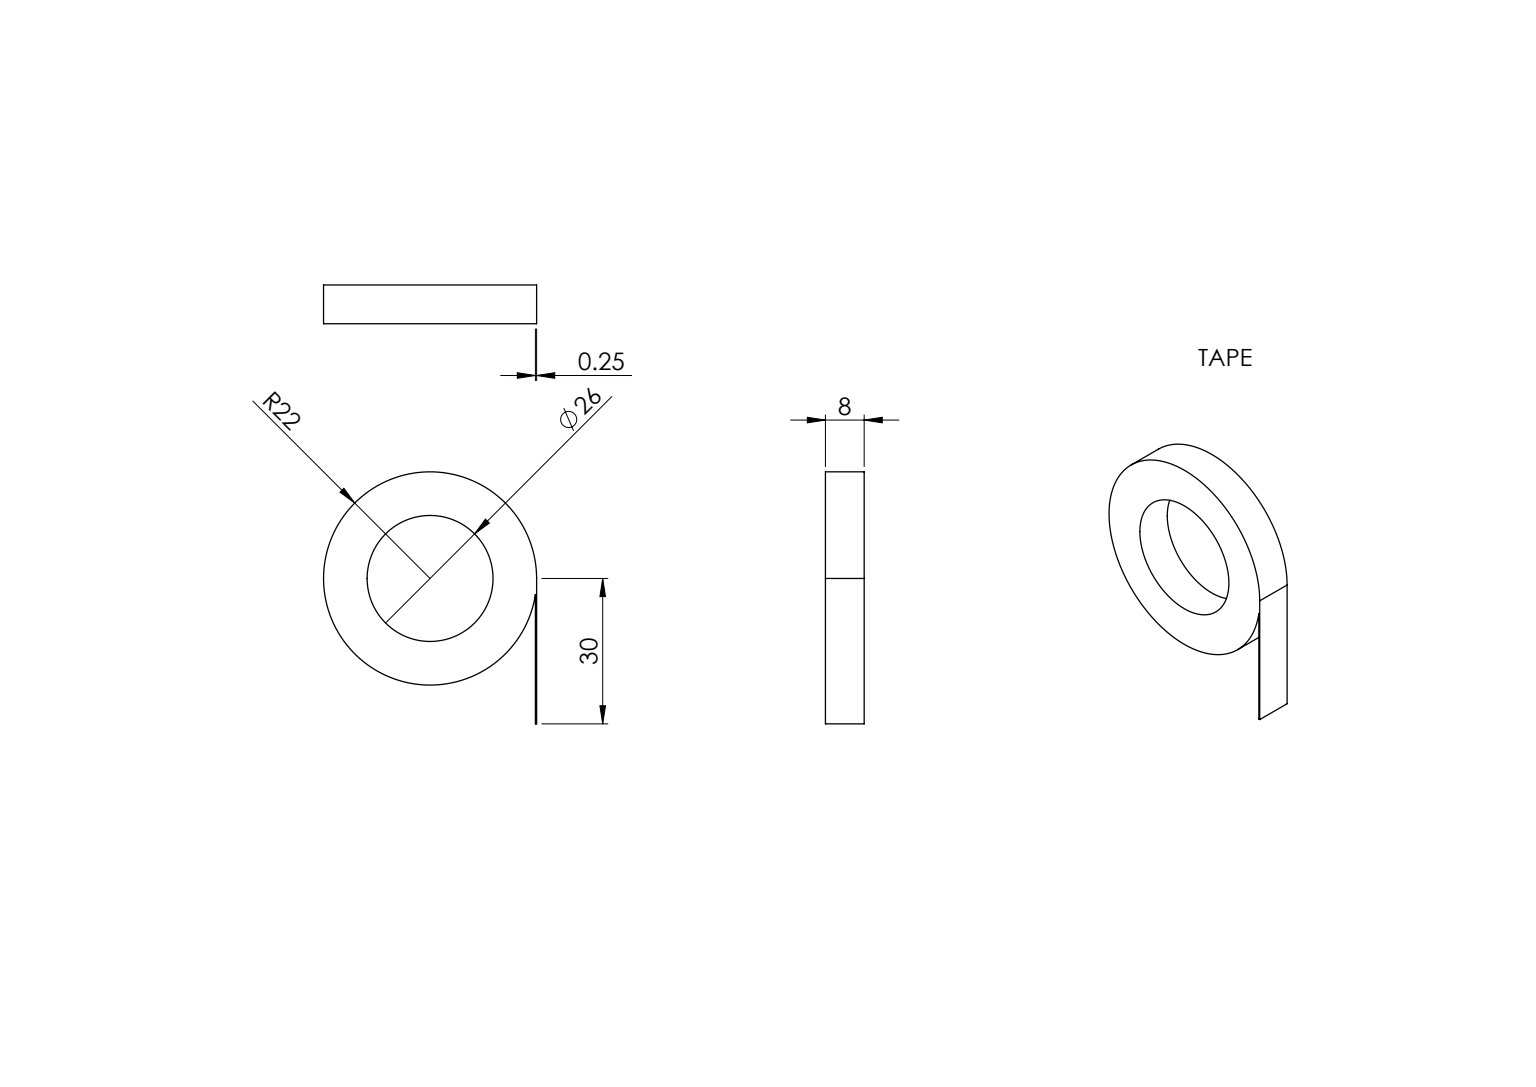
ISO-10303-21;
HEADER;
FILE_DESCRIPTION (('STEP AP214'),
    '1' );
FILE_NAME ('tape.step',
    '2026-10-23T14:45:25',
    ( '' ),
    ( '' ),
    'SwSTEP 2.0',
    'SolidWorks 2026',
    '' );
FILE_SCHEMA (( 'AUTOMOTIVE_DESIGN' ));
ENDSEC;

DATA;
#10=FACE_OUTER_BOUND ( 'NONE', #593, .T. ) ;
#25=LINE ( 'NONE', #396, #4267 ) ;
#41=DIRECTION ( 'NONE',  ( -0.000000000000000000, -0.000000000000000000, 1.000000000000000000 ) ) ;
#112=FACE_OUTER_BOUND ( 'NONE', #2425, .T. ) ;
#144=AXIS2_PLACEMENT_3D ( 'NONE', #2084, #4329, #2630 ) ;
#147=VECTOR ( 'NONE', #3798, 1000.000000000000000 ) ;
#160=DIRECTION ( 'NONE',  ( -1.000000000000000000, 1.156482317317871478E-16, 0.000000000000000000 ) ) ;
#169=FILL_AREA_STYLE ('',( #1465 ) ) ;
#177=PRODUCT_DEFINITION ( 'UNKNOWN', '', #2504, #5623 ) ;
#186=VERTEX_POINT ( 'NONE', #5039 ) ;
#263=FACE_OUTER_BOUND ( 'NONE', #5640, .T. ) ;
#276=VERTEX_POINT ( 'NONE', #4778 ) ;
#281=CARTESIAN_POINT ( 'NONE',  ( 21.74999999999999645, -30.00000000000000000, 4.000000000000001776 ) ) ;
#283=CARTESIAN_POINT ( 'NONE',  ( 0.000000000000000000, 0.000000000000000000, 0.000000000000000000 ) ) ;
#300=VERTEX_POINT ( 'NONE', #812 ) ;
#317=CARTESIAN_POINT ( 'NONE',  ( 21.74999999999999645, -30.00000000000000000, 4.000000000000001776 ) ) ;
#322=AXIS2_PLACEMENT_3D ( 'NONE', #2249, #3206, #3094 ) ;
#341=DIRECTION ( 'NONE',  ( -0.000000000000000000, -0.000000000000000000, 1.000000000000000000 ) ) ;
#377=ORIENTED_EDGE ( 'NONE', *, *, #2965, .T. ) ;
#391=PRODUCT_CONTEXT ( 'NONE', #2359, 'mechanical' ) ;
#396=CARTESIAN_POINT ( 'NONE',  ( 22.00000000000000000, 0.000000000000000000, 4.000000000000001776 ) ) ;
#443=EDGE_LOOP ( 'NONE', ( #3408, #675, #377, #4015 ) ) ;
#514=DIRECTION ( 'NONE',  ( -1.156482317317871478E-16, -1.000000000000000000, 0.000000000000000000 ) ) ;
#593=EDGE_LOOP ( 'NONE', ( #4807, #5299, #2400, #5252 ) ) ;
#599=SURFACE_STYLE_USAGE ( .BOTH. , #3222 ) ;
#602=ORIENTED_EDGE ( 'NONE', *, *, #3162, .F. ) ;
#606=CIRCLE ( 'NONE', #4005, 22.00000000000000000 ) ;
#675=ORIENTED_EDGE ( 'NONE', *, *, #3739, .T. ) ;
#687=EDGE_CURVE ( 'NONE', #2844, #5686, #1361, .T. ) ;
#701=AXIS2_PLACEMENT_3D ( 'NONE', #1249, #817, #1709 ) ;
#717=VECTOR ( 'NONE', #3845, 1000.000000000000000 ) ;
#720=AXIS2_PLACEMENT_3D ( 'NONE', #2496, #3826, #4630 ) ;
#723=CARTESIAN_POINT ( 'NONE',  ( 0.000000000000000000, 0.000000000000000000, 12.00000000000000000 ) ) ;
#764=ADVANCED_FACE ( 'NONE', ( #112 ), #4631, .F. ) ;
#772=LINE ( 'NONE', #281, #3560 ) ;
#809=CARTESIAN_POINT ( 'NONE',  ( 21.75000000000000000, -3.307189138830739061, -58.22539674441618018 ) ) ;
#812=CARTESIAN_POINT ( 'NONE',  ( 21.99999999999999645, -30.00000000000000000, 4.000000000000001776 ) ) ;
#817=DIRECTION ( 'NONE',  ( 0.000000000000000000, 0.000000000000000000, -1.000000000000000000 ) ) ;
#829=SHAPE_DEFINITION_REPRESENTATION ( #2987, #1911 ) ;
#843=ORIENTED_EDGE ( 'NONE', *, *, #1114, .T. ) ;
#861=LINE ( 'NONE', #5267, #1138 ) ;
#905=CARTESIAN_POINT ( 'NONE',  ( -13.00000000000000178, 1.592040838891559293E-15, -58.22539674441618018 ) ) ;
#907=EDGE_LOOP ( 'NONE', ( #5557, #3894 ) ) ;
#947=CARTESIAN_POINT ( 'NONE',  ( -13.00000000000000178, 1.592040838891559293E-15, 12.00000000000000000 ) ) ;
#949=CARTESIAN_POINT ( 'NONE',  ( 21.74999999999999645, -30.00000000000000000, 12.00000000000000000 ) ) ;
#998=ADVANCED_FACE ( 'NONE', ( #2029 ), #2922, .F. ) ;
#1031=DIRECTION ( 'NONE',  ( -0.000000000000000000, -0.000000000000000000, 1.000000000000000000 ) ) ;
#1035=ORIENTED_EDGE ( 'NONE', *, *, #4653, .T. ) ;
#1070=DIRECTION ( 'NONE',  ( 0.000000000000000000, -0.000000000000000000, -1.000000000000000000 ) ) ;
#1094=EDGE_CURVE ( 'NONE', #300, #5686, #5596, .T. ) ;
#1114=EDGE_CURVE ( 'NONE', #5601, #276, #2089, .T. ) ;
#1138=VECTOR ( 'NONE', #3169, 1000.000000000000000 ) ;
#1148=AXIS2_PLACEMENT_3D ( 'NONE', #5005, #4577, #2387 ) ;
#1173=ORIENTED_EDGE ( 'NONE', *, *, #1220, .F. ) ;
#1220=EDGE_CURVE ( 'NONE', #186, #300, #4785, .T. ) ;
#1249=CARTESIAN_POINT ( 'NONE',  ( 0.000000000000000000, 0.000000000000000000, 4.000000000000000000 ) ) ;
#1282=FACE_OUTER_BOUND ( 'NONE', #5045, .T. ) ;
#1299=DIRECTION ( 'NONE',  ( 0.000000000000000000, 0.000000000000000000, -1.000000000000000000 ) ) ;
#1311=CARTESIAN_POINT ( 'NONE',  ( 13.00000000000000178, 0.000000000000000000, -58.22539674441618018 ) ) ;
#1312=MECHANICAL_DESIGN_GEOMETRIC_PRESENTATION_REPRESENTATION('',(#4977),#2871);
#1330=DIRECTION ( 'NONE',  ( -1.156482317317871725E-16, -1.000000000000000000, 0.000000000000000000 ) ) ;
#1333=VERTEX_POINT ( 'NONE', #5245 ) ;
#1336=AXIS2_PLACEMENT_3D ( 'NONE', #283, #2997, #5213 ) ;
#1340=LINE ( 'NONE', #1311, #1873 ) ;
#1357=CIRCLE ( 'NONE', #1726, 13.00000000000000178 ) ;
#1361=LINE ( 'NONE', #1901, #4114 ) ;
#1397=VERTEX_POINT ( 'NONE', #949 ) ;
#1445=PLANE ( 'NONE',  #1148 ) ;
#1465=FILL_AREA_STYLE_COLOUR ( '', #3791 ) ;
#1500=CIRCLE ( 'NONE', #2792, 13.00000000000000178 ) ;
#1512=APPLICATION_CONTEXT ( 'automotive_design' ) ;
#1536=AXIS2_PLACEMENT_3D ( 'NONE', #3659, #1031, #3741 ) ;
#1570=EDGE_LOOP ( 'NONE', ( #4840, #1897, #4181, #4871 ) ) ;
#1571=DIRECTION ( 'NONE',  ( -1.156482317317871478E-16, -1.000000000000000000, 0.000000000000000000 ) ) ;
#1575=ORIENTED_EDGE ( 'NONE', *, *, #4653, .F. ) ;
#1662=LINE ( 'NONE', #5630, #4817 ) ;
#1670=DIRECTION ( 'NONE',  ( 0.000000000000000000, 0.000000000000000000, -1.000000000000000000 ) ) ;
#1685=ORIENTED_EDGE ( 'NONE', *, *, #4947, .F. ) ;
#1709=DIRECTION ( 'NONE',  ( -1.000000000000000000, 0.000000000000000000, -0.000000000000000000 ) ) ;
#1726=AXIS2_PLACEMENT_3D ( 'NONE', #723, #5172, #5123 ) ;
#1730=DIRECTION ( 'NONE',  ( -1.000000000000000000, 0.000000000000000000, 0.000000000000000000 ) ) ;
#1780=EDGE_CURVE ( 'NONE', #4073, #2517, #1357, .T. ) ;
#1796=AXIS2_PLACEMENT_3D ( 'NONE', #3149, #3516, #4496 ) ;
#1821=FACE_OUTER_BOUND ( 'NONE', #443, .T. ) ;
#1842=EDGE_CURVE ( 'NONE', #186, #1397, #772, .T. ) ;
#1844=ADVANCED_FACE ( 'NONE', ( #2069 ), #3446, .F. ) ;
#1873=VECTOR ( 'NONE', #3100, 1000.000000000000000 ) ;
#1897=ORIENTED_EDGE ( 'NONE', *, *, #4420, .T. ) ;
#1901=CARTESIAN_POINT ( 'NONE',  ( 22.00000000000000000, 0.000000000000000000, 12.00000000000000000 ) ) ;
#1903=AXIS2_PLACEMENT_3D ( 'NONE', #5424, #160, #1571 ) ;
#1911=SHAPE_REPRESENTATION ( 'tape', ( #1336 ), #5538 ) ;
#1976=ORIENTED_EDGE ( 'NONE', *, *, #4934, .T. ) ;
#1993=DIRECTION ( 'NONE',  ( 0.000000000000000000, -1.000000000000000000, 0.000000000000000000 ) ) ;
#2029=FACE_OUTER_BOUND ( 'NONE', #5048, .T. ) ;
#2069=FACE_OUTER_BOUND ( 'NONE', #3434, .T. ) ;
#2076=ORIENTED_EDGE ( 'NONE', *, *, #1220, .T. ) ;
#2084=CARTESIAN_POINT ( 'NONE',  ( 0.000000000000000000, 0.000000000000000000, 12.00000000000000000 ) ) ;
#2086=CARTESIAN_POINT ( 'NONE',  ( 21.99999999999999645, -30.00000000000000000, 4.000000000000001776 ) ) ;
#2089=CIRCLE ( 'NONE', #3556, 13.00000000000000178 ) ;
#2171=CARTESIAN_POINT ( 'NONE',  ( 21.74999999999999645, -30.00000000000000000, 4.000000000000001776 ) ) ;
#2192=ORIENTED_EDGE ( 'NONE', *, *, #3796, .T. ) ;
#2240=DIRECTION ( 'NONE',  ( -0.000000000000000000, -0.000000000000000000, 1.000000000000000000 ) ) ;
#2249=CARTESIAN_POINT ( 'NONE',  ( 0.000000000000000000, 0.000000000000000000, -58.22539674441618018 ) ) ;
#2252=ORIENTED_EDGE ( 'NONE', *, *, #1780, .F. ) ;
#2268=CARTESIAN_POINT ( 'NONE',  ( 13.00000000000000178, 0.000000000000000000, 12.00000000000000000 ) ) ;
#2279=ORIENTED_EDGE ( 'NONE', *, *, #4046, .F. ) ;
#2288=ADVANCED_FACE ( 'NONE', ( #263 ), #4266, .T. ) ;
#2327=MECHANICAL_DESIGN_GEOMETRIC_PRESENTATION_REPRESENTATION('',(#5638),#3526);
#2359=APPLICATION_CONTEXT ( 'automotive_design' ) ;
#2381=PRESENTATION_STYLE_ASSIGNMENT (( #599 ) ) ;
#2386=DIRECTION ( 'NONE',  ( -1.156482317317871478E-16, -1.000000000000000000, 0.000000000000000000 ) ) ;
#2387=DIRECTION ( 'NONE',  ( -1.000000000000000000, 0.000000000000000000, -0.000000000000000000 ) ) ;
#2400=ORIENTED_EDGE ( 'NONE', *, *, #1842, .T. ) ;
#2405=EDGE_LOOP ( 'NONE', ( #2279, #4961 ) ) ;
#2425=EDGE_LOOP ( 'NONE', ( #3605, #1035, #602, #2829 ) ) ;
#2477=DIRECTION ( 'NONE',  ( -1.000000000000000000, 0.000000000000000000, 0.000000000000000000 ) ) ;
#2496=CARTESIAN_POINT ( 'NONE',  ( 0.000000000000000000, 0.000000000000000000, -58.22539674441618018 ) ) ;
#2504=PRODUCT_DEFINITION_FORMATION_WITH_SPECIFIED_SOURCE ( 'ANY', '', #2846, .NOT_KNOWN. ) ;
#2509=PLANE ( 'NONE',  #701 ) ;
#2517=VERTEX_POINT ( 'NONE', #2268 ) ;
#2546=CLOSED_SHELL ( 'NONE', ( #764, #3249, #5603, #1844, #3057, #3313, #998, #2288 ) ) ;
#2561=LINE ( 'NONE', #809, #147 ) ;
#2609=DIRECTION ( 'NONE',  ( -1.156482317317871725E-16, -1.000000000000000000, 0.000000000000000000 ) ) ;
#2630=DIRECTION ( 'NONE',  ( -1.000000000000000000, 0.000000000000000000, 0.000000000000000000 ) ) ;
#2769=CYLINDRICAL_SURFACE ( 'NONE', #322, 22.00000000000000000 ) ;
#2792=AXIS2_PLACEMENT_3D ( 'NONE', #4862, #1299, #1730 ) ;
#2795=VECTOR ( 'NONE', #41, 1000.000000000000000 ) ;
#2812=ORIENTED_EDGE ( 'NONE', *, *, #1842, .F. ) ;
#2818=SHAPE_REPRESENTATION_RELATIONSHIP ( 'NONE' , 'NONE' ,  #1911, #5006 ) ;
#2825=CARTESIAN_POINT ( 'NONE',  ( -13.00000000000000178, 1.592040838891559293E-15, 4.000000000000003553 ) ) ;
#2829=ORIENTED_EDGE ( 'NONE', *, *, #4629, .F. ) ;
#2837=CARTESIAN_POINT ( 'NONE',  ( 22.00000000000000000, 0.000000000000000000, 12.00000000000000000 ) ) ;
#2844=VERTEX_POINT ( 'NONE', #2837 ) ;
#2846=PRODUCT ( 'tape', 'tape', '', ( #391 ) ) ;
#2871=( GEOMETRIC_REPRESENTATION_CONTEXT ( 3 ) GLOBAL_UNCERTAINTY_ASSIGNED_CONTEXT ( ( #5500 ) ) GLOBAL_UNIT_ASSIGNED_CONTEXT ( ( #5407, #4569, #3701 ) ) REPRESENTATION_CONTEXT ( 'NONE', 'WORKASPACE' ) );
#2922=PLANE ( 'NONE',  #1903 ) ;
#2965=EDGE_CURVE ( 'NONE', #5441, #2844, #3091, .T. ) ;
#2987=PRODUCT_DEFINITION_SHAPE ( 'NONE', 'NONE',  #177 ) ;
#2997=DIRECTION ( 'NONE',  ( 0.000000000000000000, 0.000000000000000000, 1.000000000000000000 ) ) ;
#3057=ADVANCED_FACE ( 'NONE', ( #1282, #4808 ), #2509, .T. ) ;
#3091=CIRCLE ( 'NONE', #5660, 22.00000000000000000 ) ;
#3094=DIRECTION ( 'NONE',  ( 1.000000000000000000, 0.000000000000000000, 0.000000000000000000 ) ) ;
#3100=DIRECTION ( 'NONE',  ( -0.000000000000000000, -0.000000000000000000, 1.000000000000000000 ) ) ;
#3113=LINE ( 'NONE', #3569, #3529 ) ;
#3124=ORIENTED_EDGE ( 'NONE', *, *, #687, .T. ) ;
#3149=CARTESIAN_POINT ( 'NONE',  ( 21.75000000000000000, 2.891205793294679929E-17, 4.000000000000001776 ) ) ;
#3162=EDGE_CURVE ( 'NONE', #2517, #4073, #5564, .T. ) ;
#3169=DIRECTION ( 'NONE',  ( 1.000000000000000000, 0.000000000000000000, 0.000000000000000000 ) ) ;
#3205=FACE_BOUND ( 'NONE', #907, .T. ) ;
#3206=DIRECTION ( 'NONE',  ( -0.000000000000000000, -0.000000000000000000, 1.000000000000000000 ) ) ;
#3222=SURFACE_SIDE_STYLE ('',( #5057 ) ) ;
#3247=( NAMED_UNIT ( * ) PLANE_ANGLE_UNIT ( ) SI_UNIT ( $, .RADIAN. ) );
#3249=ADVANCED_FACE ( 'NONE', ( #1821 ), #2769, .T. ) ;
#3313=ADVANCED_FACE ( 'NONE', ( #10 ), #3578, .T. ) ;
#3343=VECTOR ( 'NONE', #1330, 1000.000000000000000 ) ;
#3408=ORIENTED_EDGE ( 'NONE', *, *, #3796, .F. ) ;
#3411=CARTESIAN_POINT ( 'NONE',  ( 0.000000000000000000, 0.000000000000000000, 4.000000000000003553 ) ) ;
#3434=EDGE_LOOP ( 'NONE', ( #1575, #843, #4249, #2252 ) ) ;
#3446=CYLINDRICAL_SURFACE ( 'NONE', #720, 13.00000000000000178 ) ;
#3466=DIRECTION ( 'NONE',  ( 0.000000000000000000, 0.000000000000000000, -1.000000000000000000 ) ) ;
#3470=LINE ( 'NONE', #905, #2795 ) ;
#3516=DIRECTION ( 'NONE',  ( -1.000000000000000000, 1.156482317317871725E-16, 0.000000000000000000 ) ) ;
#3526=( GEOMETRIC_REPRESENTATION_CONTEXT ( 3 ) GLOBAL_UNCERTAINTY_ASSIGNED_CONTEXT ( ( #4493 ) ) GLOBAL_UNIT_ASSIGNED_CONTEXT ( ( #5249, #4806, #4384 ) ) REPRESENTATION_CONTEXT ( 'NONE', 'WORKASPACE' ) );
#3529=VECTOR ( 'NONE', #514, 1000.000000000000000 ) ;
#3556=AXIS2_PLACEMENT_3D ( 'NONE', #3411, #3466, #5163 ) ;
#3560=VECTOR ( 'NONE', #341, 1000.000000000000000 ) ;
#3568=UNCERTAINTY_MEASURE_WITH_UNIT (LENGTH_MEASURE( 1.000000000000000082E-05 ), #3995, 'distance_accuracy_value', 'NONE');
#3569=CARTESIAN_POINT ( 'NONE',  ( 22.00000000000000000, 0.000000000000000000, 4.000000000000001776 ) ) ;
#3578=PLANE ( 'NONE',  #1796 ) ;
#3605=ORIENTED_EDGE ( 'NONE', *, *, #4046, .T. ) ;
#3623=VERTEX_POINT ( 'NONE', #5064 ) ;
#3659=CARTESIAN_POINT ( 'NONE',  ( 0.000000000000000000, 0.000000000000000000, -58.22539674441618018 ) ) ;
#3701=( NAMED_UNIT ( * ) SI_UNIT ( $, .STERADIAN. ) SOLID_ANGLE_UNIT ( ) );
#3739=EDGE_CURVE ( 'NONE', #1333, #5441, #2561, .T. ) ;
#3741=DIRECTION ( 'NONE',  ( 1.000000000000000000, 0.000000000000000000, 0.000000000000000000 ) ) ;
#3754=DIRECTION ( 'NONE',  ( -1.000000000000000000, 0.000000000000000000, 0.000000000000000000 ) ) ;
#3781=ORIENTED_EDGE ( 'NONE', *, *, #4072, .F. ) ;
#3791=COLOUR_RGB ( '',0.8941176470588234615, 0.8941176470588234615, 0.8941176470588234615 ) ;
#3796=EDGE_CURVE ( 'NONE', #1333, #3623, #606, .T. ) ;
#3798=DIRECTION ( 'NONE',  ( -0.000000000000000000, -0.000000000000000000, 1.000000000000000000 ) ) ;
#3809=CARTESIAN_POINT ( 'NONE',  ( 0.000000000000000000, 0.000000000000000000, 12.00000000000000000 ) ) ;
#3826=DIRECTION ( 'NONE',  ( -0.000000000000000000, -0.000000000000000000, 1.000000000000000000 ) ) ;
#3845=DIRECTION ( 'NONE',  ( -0.000000000000000000, -0.000000000000000000, 1.000000000000000000 ) ) ;
#3864=CARTESIAN_POINT ( 'NONE',  ( 21.75000000000000000, 2.891205793294679929E-17, 12.00000000000000000 ) ) ;
#3894=ORIENTED_EDGE ( 'NONE', *, *, #1780, .T. ) ;
#3927=DIRECTION ( 'NONE',  ( 1.000000000000000000, 0.000000000000000000, 0.000000000000000000 ) ) ;
#3995=( LENGTH_UNIT ( ) NAMED_UNIT ( * ) SI_UNIT ( .MILLI., .METRE. ) );
#3998=AXIS2_PLACEMENT_3D ( 'NONE', #317, #1993, #1070 ) ;
#4005=AXIS2_PLACEMENT_3D ( 'NONE', #4293, #1670, #2477 ) ;
#4015=ORIENTED_EDGE ( 'NONE', *, *, #4934, .F. ) ;
#4046=EDGE_CURVE ( 'NONE', #276, #5601, #1500, .T. ) ;
#4072=EDGE_CURVE ( 'NONE', #1397, #5686, #861, .T. ) ;
#4073=VERTEX_POINT ( 'NONE', #947 ) ;
#4083=( NAMED_UNIT ( * ) SI_UNIT ( $, .STERADIAN. ) SOLID_ANGLE_UNIT ( ) );
#4114=VECTOR ( 'NONE', #2386, 1000.000000000000000 ) ;
#4132=ORIENTED_EDGE ( 'NONE', *, *, #1094, .F. ) ;
#4147=FACE_OUTER_BOUND ( 'NONE', #1570, .T. ) ;
#4181=ORIENTED_EDGE ( 'NONE', *, *, #4072, .T. ) ;
#4189=DIRECTION ( 'NONE',  ( 0.000000000000000000, 0.000000000000000000, -1.000000000000000000 ) ) ;
#4249=ORIENTED_EDGE ( 'NONE', *, *, #4629, .T. ) ;
#4266=PLANE ( 'NONE',  #3998 ) ;
#4267=VECTOR ( 'NONE', #2240, 1000.000000000000000 ) ;
#4293=CARTESIAN_POINT ( 'NONE',  ( 0.000000000000000000, 0.000000000000000000, 4.000000000000003553 ) ) ;
#4329=DIRECTION ( 'NONE',  ( 0.000000000000000000, 0.000000000000000000, -1.000000000000000000 ) ) ;
#4384=( NAMED_UNIT ( * ) SI_UNIT ( $, .STERADIAN. ) SOLID_ANGLE_UNIT ( ) );
#4420=EDGE_CURVE ( 'NONE', #5441, #1397, #5676, .T. ) ;
#4482=MANIFOLD_SOLID_BREP ( 'Extrude-Thin2', #2546 ) ;
#4493=UNCERTAINTY_MEASURE_WITH_UNIT (LENGTH_MEASURE( 1.000000000000000082E-05 ), #5249, 'distance_accuracy_value', 'NONE');
#4496=DIRECTION ( 'NONE',  ( -1.156482317317871725E-16, -1.000000000000000000, 0.000000000000000000 ) ) ;
#4569=( NAMED_UNIT ( * ) PLANE_ANGLE_UNIT ( ) SI_UNIT ( $, .RADIAN. ) );
#4577=DIRECTION ( 'NONE',  ( 0.000000000000000000, 0.000000000000000000, -1.000000000000000000 ) ) ;
#4629=EDGE_CURVE ( 'NONE', #276, #2517, #1340, .T. ) ;
#4630=DIRECTION ( 'NONE',  ( 1.000000000000000000, 0.000000000000000000, 0.000000000000000000 ) ) ;
#4631=CYLINDRICAL_SURFACE ( 'NONE', #1536, 13.00000000000000178 ) ;
#4653=EDGE_CURVE ( 'NONE', #5601, #4073, #3470, .T. ) ;
#4778=CARTESIAN_POINT ( 'NONE',  ( 13.00000000000000178, 0.000000000000000000, 4.000000000000003553 ) ) ;
#4785=LINE ( 'NONE', #2171, #5669 ) ;
#4806=( NAMED_UNIT ( * ) PLANE_ANGLE_UNIT ( ) SI_UNIT ( $, .RADIAN. ) );
#4807=ORIENTED_EDGE ( 'NONE', *, *, #3739, .F. ) ;
#4808=FACE_BOUND ( 'NONE', #2405, .T. ) ;
#4817=VECTOR ( 'NONE', #2609, 1000.000000000000000 ) ;
#4840=ORIENTED_EDGE ( 'NONE', *, *, #2965, .F. ) ;
#4862=CARTESIAN_POINT ( 'NONE',  ( 0.000000000000000000, 0.000000000000000000, 4.000000000000003553 ) ) ;
#4871=ORIENTED_EDGE ( 'NONE', *, *, #687, .F. ) ;
#4934=EDGE_CURVE ( 'NONE', #3623, #2844, #25, .T. ) ;
#4947=EDGE_CURVE ( 'NONE', #3623, #300, #3113, .T. ) ;
#4952=CARTESIAN_POINT ( 'NONE',  ( 21.99999999999999645, -30.00000000000000000, 12.00000000000000000 ) ) ;
#4961=ORIENTED_EDGE ( 'NONE', *, *, #1114, .F. ) ;
#4977=STYLED_ITEM ( 'NONE', ( #2381 ), #5006 ) ;
#5005=CARTESIAN_POINT ( 'NONE',  ( 0.000000000000000000, 0.000000000000000000, 12.00000000000000000 ) ) ;
#5006=ADVANCED_BREP_SHAPE_REPRESENTATION ( '', ( #4482, #1336 ), #5538 ) ;
#5039=CARTESIAN_POINT ( 'NONE',  ( 21.74999999999999645, -30.00000000000000000, 4.000000000000001776 ) ) ;
#5045=EDGE_LOOP ( 'NONE', ( #2192, #5116, #1173, #5471 ) ) ;
#5048=EDGE_LOOP ( 'NONE', ( #3124, #4132, #1685, #1976 ) ) ;
#5057=SURFACE_STYLE_FILL_AREA ( #169 ) ;
#5064=CARTESIAN_POINT ( 'NONE',  ( 22.00000000000000000, -2.544261098099317203E-15, 4.000000000000003553 ) ) ;
#5116=ORIENTED_EDGE ( 'NONE', *, *, #4947, .T. ) ;
#5123=DIRECTION ( 'NONE',  ( -1.000000000000000000, 0.000000000000000000, 0.000000000000000000 ) ) ;
#5163=DIRECTION ( 'NONE',  ( -1.000000000000000000, 0.000000000000000000, 0.000000000000000000 ) ) ;
#5172=DIRECTION ( 'NONE',  ( 0.000000000000000000, 0.000000000000000000, -1.000000000000000000 ) ) ;
#5213=DIRECTION ( 'NONE',  ( 1.000000000000000000, 0.000000000000000000, 0.000000000000000000 ) ) ;
#5224=ORIENTED_EDGE ( 'NONE', *, *, #1094, .T. ) ;
#5245=CARTESIAN_POINT ( 'NONE',  ( 21.75000000000000000, -3.307189138830739061, 4.000000000000001776 ) ) ;
#5249=( LENGTH_UNIT ( ) NAMED_UNIT ( * ) SI_UNIT ( .MILLI., .METRE. ) );
#5252=ORIENTED_EDGE ( 'NONE', *, *, #4420, .F. ) ;
#5267=CARTESIAN_POINT ( 'NONE',  ( 21.74999999999999645, -30.00000000000000000, 12.00000000000000000 ) ) ;
#5299=ORIENTED_EDGE ( 'NONE', *, *, #5501, .T. ) ;
#5407=( LENGTH_UNIT ( ) NAMED_UNIT ( * ) SI_UNIT ( .MILLI., .METRE. ) );
#5424=CARTESIAN_POINT ( 'NONE',  ( 22.00000000000000000, 0.000000000000000000, 4.000000000000001776 ) ) ;
#5441=VERTEX_POINT ( 'NONE', #5576 ) ;
#5471=ORIENTED_EDGE ( 'NONE', *, *, #5501, .F. ) ;
#5500=UNCERTAINTY_MEASURE_WITH_UNIT (LENGTH_MEASURE( 1.000000000000000082E-05 ), #5407, 'distance_accuracy_value', 'NONE');
#5501=EDGE_CURVE ( 'NONE', #1333, #186, #1662, .T. ) ;
#5538=( GEOMETRIC_REPRESENTATION_CONTEXT ( 3 ) GLOBAL_UNCERTAINTY_ASSIGNED_CONTEXT ( ( #3568 ) ) GLOBAL_UNIT_ASSIGNED_CONTEXT ( ( #3995, #3247, #4083 ) ) REPRESENTATION_CONTEXT ( 'NONE', 'WORKASPACE' ) );
#5557=ORIENTED_EDGE ( 'NONE', *, *, #3162, .T. ) ;
#5564=CIRCLE ( 'NONE', #144, 13.00000000000000178 ) ;
#5576=CARTESIAN_POINT ( 'NONE',  ( 21.75000000000000000, -3.307189138830739061, 12.00000000000000000 ) ) ;
#5596=LINE ( 'NONE', #2086, #717 ) ;
#5601=VERTEX_POINT ( 'NONE', #2825 ) ;
#5603=ADVANCED_FACE ( 'NONE', ( #4147, #3205 ), #1445, .F. ) ;
#5623=PRODUCT_DEFINITION_CONTEXT ( 'detailed design', #1512, 'design' ) ;
#5630=CARTESIAN_POINT ( 'NONE',  ( 21.75000000000000000, 2.891205793294679929E-17, 4.000000000000001776 ) ) ;
#5638=STYLED_ITEM('',(#5716),#4482);
#5640=EDGE_LOOP ( 'NONE', ( #3781, #2812, #2076, #5224 ) ) ;
#5660=AXIS2_PLACEMENT_3D ( 'NONE', #3809, #4189, #3754 ) ;
#5669=VECTOR ( 'NONE', #3927, 1000.000000000000000 ) ;
#5676=LINE ( 'NONE', #3864, #3343 ) ;
#5686=VERTEX_POINT ( 'NONE', #4952 ) ;
#5710=COLOUR_RGB('Sky Blue',0.24,0.69,0.87);
#5711=FILL_AREA_STYLE_COLOUR('',#5710);
#5712=FILL_AREA_STYLE('',(#5711));
#5713=SURFACE_STYLE_FILL_AREA(#5712);
#5714=SURFACE_SIDE_STYLE('',(#5713));
#5715=SURFACE_STYLE_USAGE(.BOTH.,#5714);
#5716=PRESENTATION_STYLE_ASSIGNMENT((#5715));
ENDSEC;
END-ISO-10303-21;
